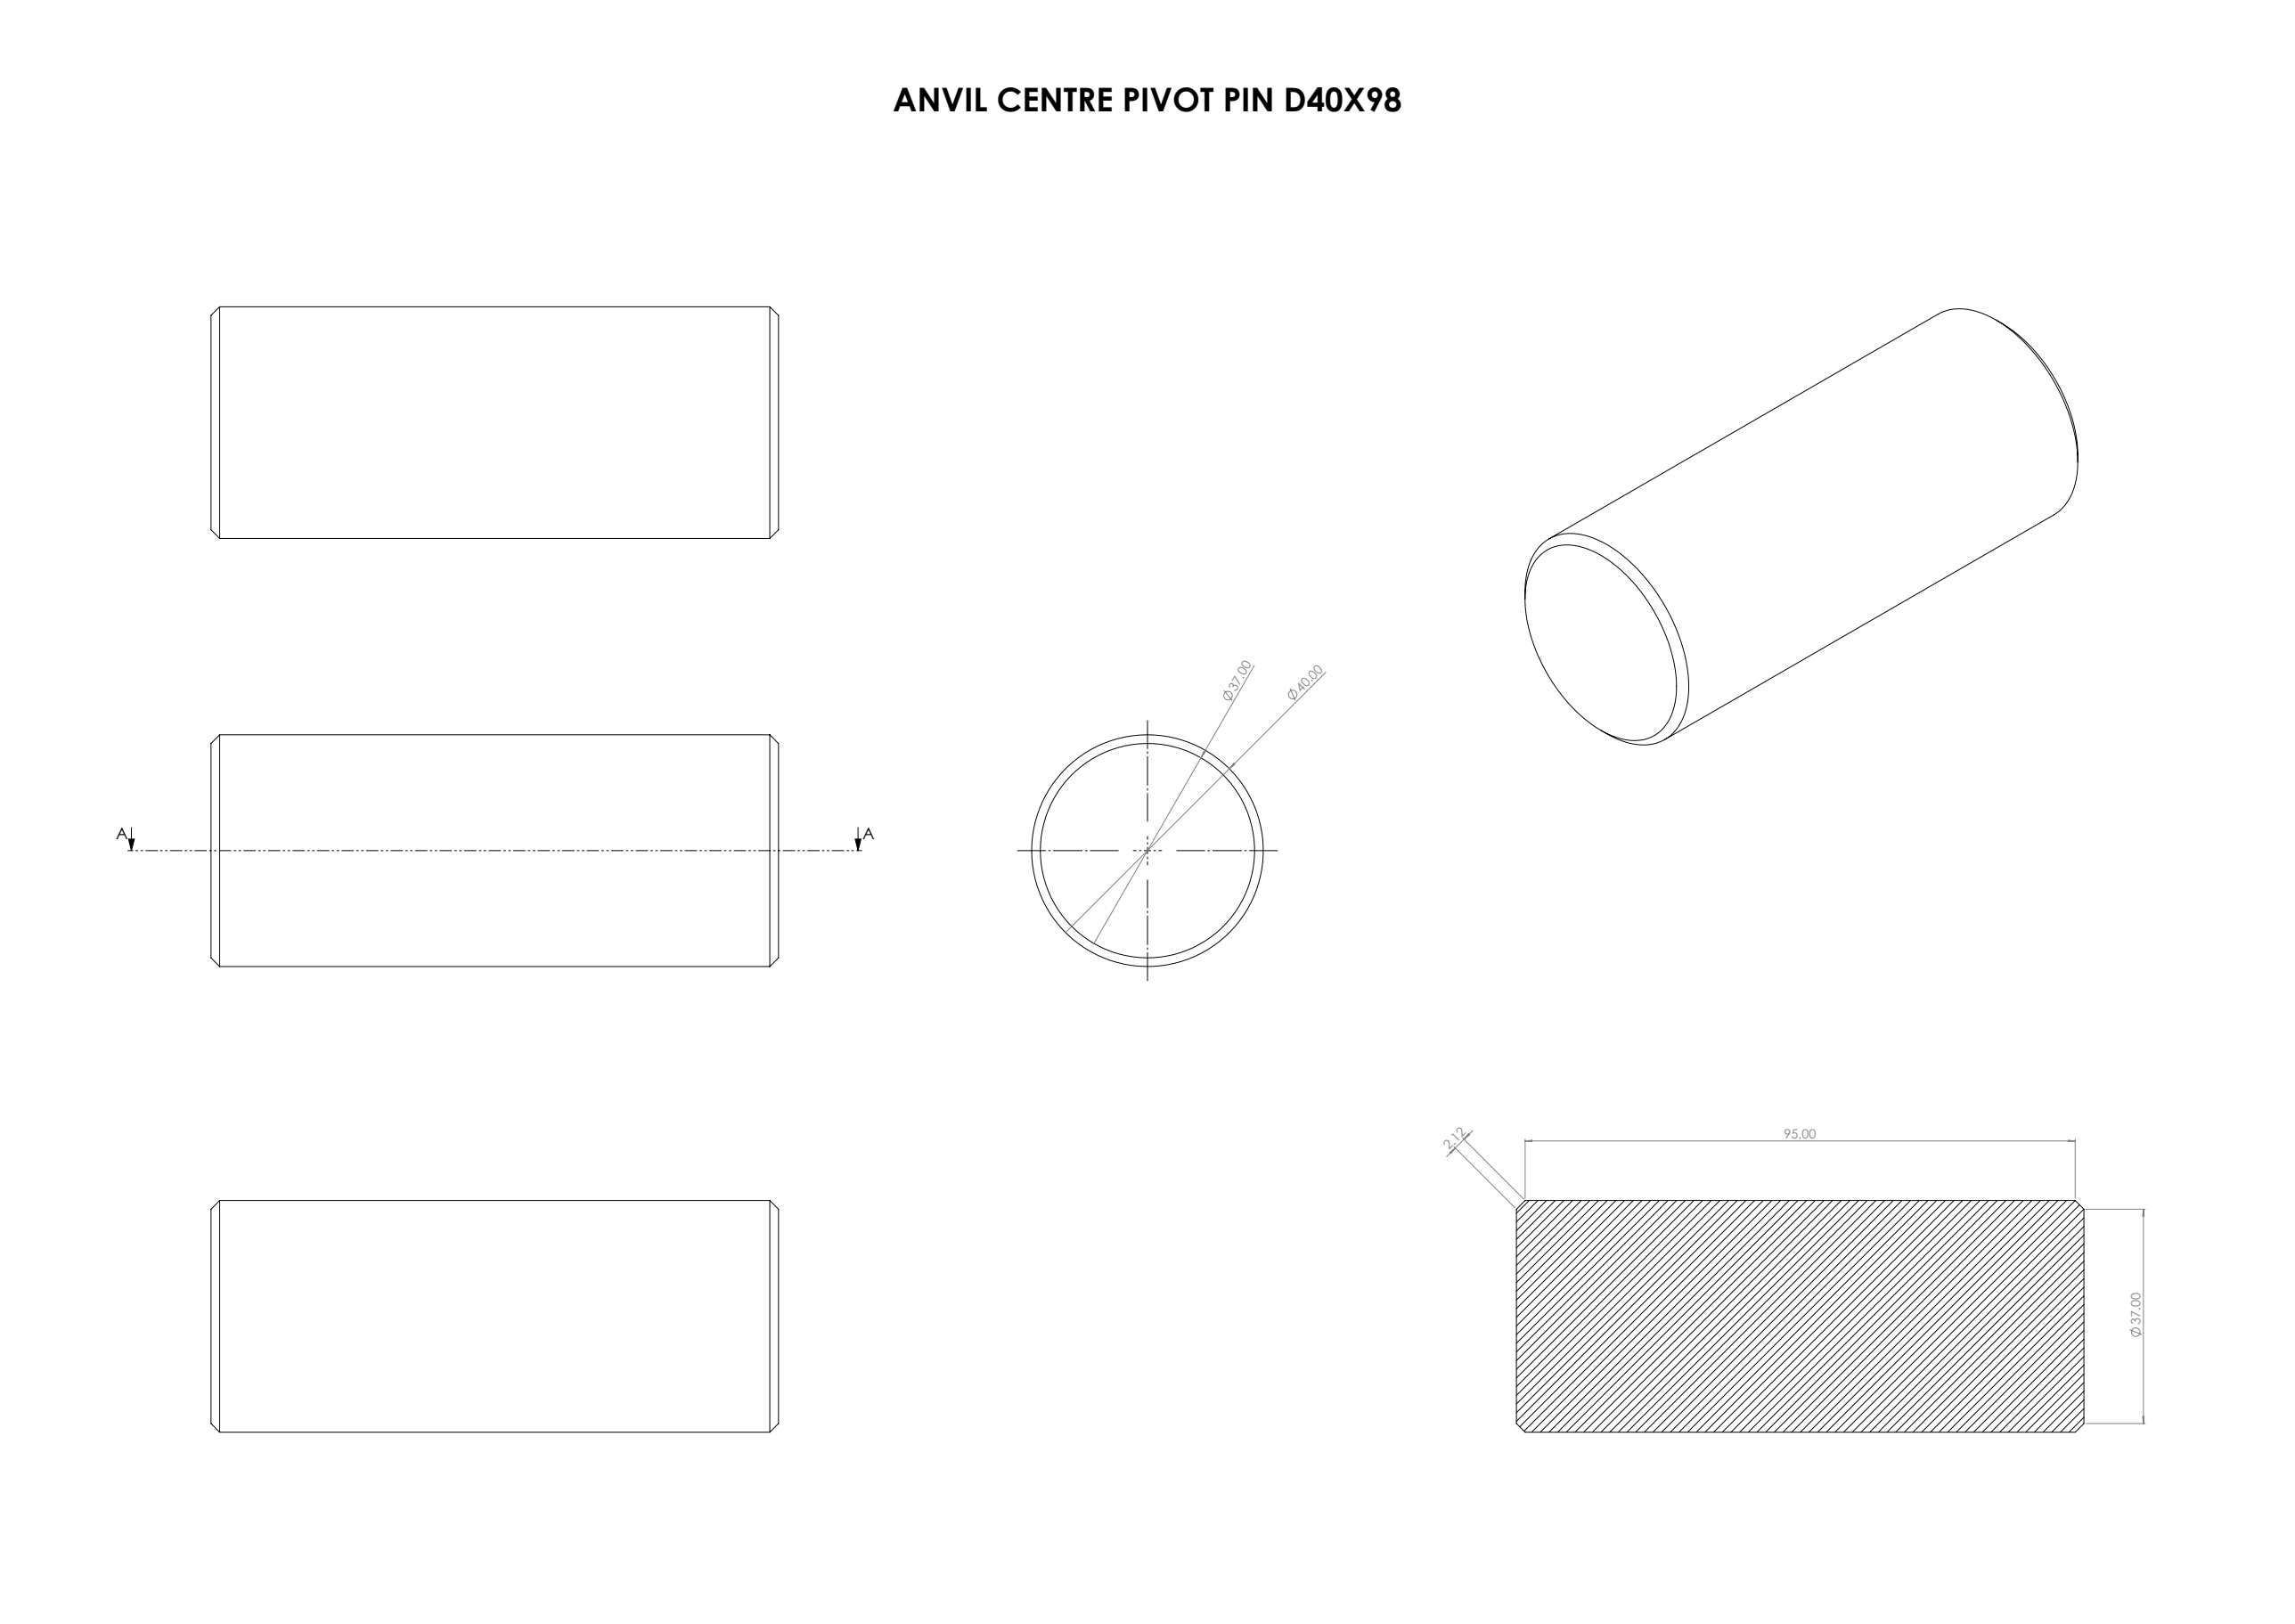
ISO-10303-21;
HEADER;
/* Generated by software containing ST-Developer
 * from STEP Tools, Inc. (www.steptools.com) 
 */

FILE_DESCRIPTION(
/* description */ (''),
/* implementation_level */ '2;1');

FILE_NAME(
/* name */ '09_Anvil_Centre_Pivot_Pin_D40x98.step',
/* time_stamp */ '2026-10-19T23:58:09-07:00',
/* author */ (''),
/* organization */ (''),
/* preprocessor_version */ 'ST-DEVELOPER v20.2',
/* originating_system */ 'Autodesk Translation Framework v15.15.0.0',
/* authorisation */ '');

FILE_SCHEMA (('AP203_CONFIGURATION_CONTROLLED_3D_DESIGN_OF_MECHANICAL_PARTS_AND_ASSEMBLIES_MIM_LF { 1 0 10303 203 3 1 4 }',
'AUTOMOTIVE_DESIGN { 1 0 10303 214 3 1 1 }','INTEGRATED_CNC_SCHEMA','MODEL_BASED_INTEGRATED_MANUFACTURING_SCHEMA',
'PROCESS_PLANNING_SCHEMA','AP242_MANAGED_MODEL_BASED_3D_ENGINEERING_MIM_LF { 1 0 10303 442 3 1 4 }'));
ENDSEC;

DATA;
#10=MECHANICAL_DESIGN_GEOMETRIC_PRESENTATION_REPRESENTATION('',(#410),#70757);
#380=SHAPE_REPRESENTATION_RELATIONSHIP('SRR','None',#70821,#395);
#395=ADVANCED_BREP_SHAPE_REPRESENTATION('',(#470),#70745);
#410=STYLED_ITEM('',(#71047),#470);
#470=MANIFOLD_SOLID_BREP('Pin',#26875);
#596=CYLINDRICAL_SURFACE('',#27394,2.);
#1761=PLANE('',#27390);
#1762=PLANE('',#27398);
#2798=FACE_OUTER_BOUND('',#4294,.T.);
#2799=FACE_OUTER_BOUND('',#4295,.T.);
#2800=FACE_OUTER_BOUND('',#4296,.T.);
#2801=FACE_OUTER_BOUND('',#4297,.T.);
#2802=FACE_OUTER_BOUND('',#4298,.T.);
#4294=EDGE_LOOP('',(#18746));
#4295=EDGE_LOOP('',(#18747,#18748,#18749,#18750));
#4296=EDGE_LOOP('',(#18751,#18752,#18753,#18754));
#4297=EDGE_LOOP('',(#18755,#18756,#18757,#18758));
#4298=EDGE_LOOP('',(#18759));
#5905=LINE('',#44061,#8402);
#5906=LINE('',#44065,#8403);
#5907=LINE('',#44069,#8404);
#8402=VECTOR('',#29942,1.925);
#8403=VECTOR('',#29947,2.);
#8404=VECTOR('',#29952,1.925);
#10766=CIRCLE('',#27391,1.85);
#10767=CIRCLE('',#27393,2.);
#10768=CIRCLE('',#27395,2.);
#10769=CIRCLE('',#27397,1.85);
#11546=VERTEX_POINT('',#44056);
#11547=VERTEX_POINT('',#44059);
#11548=VERTEX_POINT('',#44063);
#11549=VERTEX_POINT('',#44067);
#14226=EDGE_CURVE('',#11546,#11546,#10766,.T.);
#14227=EDGE_CURVE('',#11547,#11547,#10767,.T.);
#14228=EDGE_CURVE('',#11547,#11546,#5905,.T.);
#14229=EDGE_CURVE('',#11548,#11548,#10768,.T.);
#14230=EDGE_CURVE('',#11548,#11547,#5906,.T.);
#14231=EDGE_CURVE('',#11549,#11549,#10769,.T.);
#14232=EDGE_CURVE('',#11549,#11548,#5907,.T.);
#18746=ORIENTED_EDGE('',*,*,#14226,.F.);
#18747=ORIENTED_EDGE('',*,*,#14227,.F.);
#18748=ORIENTED_EDGE('',*,*,#14228,.T.);
#18749=ORIENTED_EDGE('',*,*,#14226,.T.);
#18750=ORIENTED_EDGE('',*,*,#14228,.F.);
#18751=ORIENTED_EDGE('',*,*,#14229,.F.);
#18752=ORIENTED_EDGE('',*,*,#14230,.T.);
#18753=ORIENTED_EDGE('',*,*,#14227,.T.);
#18754=ORIENTED_EDGE('',*,*,#14230,.F.);
#18755=ORIENTED_EDGE('',*,*,#14231,.F.);
#18756=ORIENTED_EDGE('',*,*,#14232,.T.);
#18757=ORIENTED_EDGE('',*,*,#14229,.T.);
#18758=ORIENTED_EDGE('',*,*,#14232,.F.);
#18759=ORIENTED_EDGE('',*,*,#14231,.T.);
#25321=CONICAL_SURFACE('',#27392,1.925,0.785398163397448);
#25322=CONICAL_SURFACE('',#27396,1.925,0.785398163397448);
#25611=ADVANCED_FACE('',(#2798),#1761,.T.);
#25612=ADVANCED_FACE('',(#2799),#25321,.T.);
#25613=ADVANCED_FACE('',(#2800),#596,.T.);
#25614=ADVANCED_FACE('',(#2801),#25322,.T.);
#25615=ADVANCED_FACE('',(#2802),#1762,.T.);
#26875=CLOSED_SHELL('',(#25611,#25612,#25613,#25614,#25615));
#27389=AXIS2_PLACEMENT_3D('',#44054,#29932,#29933);
#27390=AXIS2_PLACEMENT_3D('',#44055,#29934,#29935);
#27391=AXIS2_PLACEMENT_3D('',#44057,#29936,#29937);
#27392=AXIS2_PLACEMENT_3D('',#44058,#29938,#29939);
#27393=AXIS2_PLACEMENT_3D('',#44060,#29940,#29941);
#27394=AXIS2_PLACEMENT_3D('',#44062,#29943,#29944);
#27395=AXIS2_PLACEMENT_3D('',#44064,#29945,#29946);
#27396=AXIS2_PLACEMENT_3D('',#44066,#29948,#29949);
#27397=AXIS2_PLACEMENT_3D('',#44068,#29950,#29951);
#27398=AXIS2_PLACEMENT_3D('',#44070,#29953,#29954);
#29932=DIRECTION('axis',(0.,0.,1.));
#29933=DIRECTION('refdir',(1.,0.,0.));
#29934=DIRECTION('center_axis',(0.,0.,-1.));
#29935=DIRECTION('ref_axis',(-1.,0.,0.));
#29936=DIRECTION('center_axis',(0.,0.,1.));
#29937=DIRECTION('ref_axis',(1.,0.,0.));
#29938=DIRECTION('center_axis',(0.,0.,1.));
#29939=DIRECTION('ref_axis',(1.,0.,0.));
#29940=DIRECTION('center_axis',(0.,0.,1.));
#29941=DIRECTION('ref_axis',(1.,0.,0.));
#29942=DIRECTION('',(0.707106781186547,8.65956056235493E-17,-0.707106781186547));
#29943=DIRECTION('center_axis',(0.,0.,1.));
#29944=DIRECTION('ref_axis',(1.,0.,0.));
#29945=DIRECTION('center_axis',(0.,0.,1.));
#29946=DIRECTION('ref_axis',(1.,0.,0.));
#29947=DIRECTION('',(0.,0.,-1.));
#29948=DIRECTION('center_axis',(0.,0.,-1.));
#29949=DIRECTION('ref_axis',(1.,0.,0.));
#29950=DIRECTION('center_axis',(0.,0.,1.));
#29951=DIRECTION('ref_axis',(1.,0.,0.));
#29952=DIRECTION('',(-0.707106781186547,-8.65956056235493E-17,-0.707106781186547));
#29953=DIRECTION('center_axis',(0.,0.,1.));
#29954=DIRECTION('ref_axis',(1.,0.,0.));
#44054=CARTESIAN_POINT('',(0.,0.,0.));
#44055=CARTESIAN_POINT('Origin',(9.35,0.,5.5));
#44056=CARTESIAN_POINT('',(5.65,-2.2655965784226E-16,5.5));
#44057=CARTESIAN_POINT('Origin',(7.5,0.,5.5));
#44058=CARTESIAN_POINT('Origin',(7.5,0.,5.575));
#44059=CARTESIAN_POINT('',(5.5,-2.44929359829471E-16,5.65));
#44060=CARTESIAN_POINT('Origin',(7.5,0.,5.65));
#44061=CARTESIAN_POINT('',(5.575,-2.35744508835866E-16,5.575));
#44062=CARTESIAN_POINT('Origin',(7.5,0.,10.4));
#44063=CARTESIAN_POINT('',(5.5,-2.44929359829471E-16,15.15));
#44064=CARTESIAN_POINT('Origin',(7.5,0.,15.15));
#44065=CARTESIAN_POINT('',(5.5,-2.44929359829471E-16,10.4));
#44066=CARTESIAN_POINT('Origin',(7.5,0.,15.225));
#44067=CARTESIAN_POINT('',(5.65,-2.2655965784226E-16,15.3));
#44068=CARTESIAN_POINT('Origin',(7.5,0.,15.3));
#44069=CARTESIAN_POINT('',(5.575,-2.35744508835866E-16,15.225));
#44070=CARTESIAN_POINT('Origin',(7.5,0.,15.3));
#70728=UNCERTAINTY_MEASURE_WITH_UNIT(LENGTH_MEASURE(0.001),#70758,
'DISTANCE_ACCURACY_VALUE',
'Maximum model space distance between geometric entities at asserted c
onnectivities');
#70740=UNCERTAINTY_MEASURE_WITH_UNIT(LENGTH_MEASURE(0.001),#70758,
'DISTANCE_ACCURACY_VALUE',
'Maximum model space distance between geometric entities at asserted c
onnectivities');
#70745=(
GEOMETRIC_REPRESENTATION_CONTEXT(3)
GLOBAL_UNCERTAINTY_ASSIGNED_CONTEXT((#70728))
GLOBAL_UNIT_ASSIGNED_CONTEXT((#70758,#70760,#70761))
REPRESENTATION_CONTEXT('','3D')
);
#70757=(
GEOMETRIC_REPRESENTATION_CONTEXT(3)
GLOBAL_UNCERTAINTY_ASSIGNED_CONTEXT((#70740))
GLOBAL_UNIT_ASSIGNED_CONTEXT((#70758,#70760,#70761))
REPRESENTATION_CONTEXT('','3D')
);
#70758=(
LENGTH_UNIT()
NAMED_UNIT(*)
SI_UNIT(.CENTI.,.METRE.)
);
#70760=(
NAMED_UNIT(*)
PLANE_ANGLE_UNIT()
SI_UNIT($,.RADIAN.)
);
#70761=(
NAMED_UNIT(*)
SI_UNIT($,.STERADIAN.)
SOLID_ANGLE_UNIT()
);
#70766=SHAPE_DEFINITION_REPRESENTATION(#70782,#70821);
#70782=PRODUCT_DEFINITION_SHAPE('',$,#70838);
#70821=SHAPE_REPRESENTATION('',(#27389),#70745);
#70833=PRODUCT_DEFINITION_CONTEXT('part definition',#70883,'design');
#70838=PRODUCT_DEFINITION('2026-10-19-02-55-36-383',
'09_Anvil_Centre_Pivot_Pin_D40x98',#70854,#70833);
#70854=PRODUCT_DEFINITION_FORMATION('',$,#70889);
#70883=APPLICATION_CONTEXT(
'Core Data for Automotive Mechanical Design Process');
#70884=PRODUCT_CONTEXT('part definition',#70883,'mechanical');
#70889=PRODUCT('2026-10-19-02-55-36-383',
'09_Anvil_Centre_Pivot_Pin_D40x98',$,(#70884));
#71041=COLOUR_RGB('Grey',0.48,0.52,0.57);
#71042=FILL_AREA_STYLE_COLOUR('',#71041);
#71043=FILL_AREA_STYLE('',(#71042));
#71044=SURFACE_STYLE_FILL_AREA(#71043);
#71045=SURFACE_SIDE_STYLE('',(#71044));
#71046=SURFACE_STYLE_USAGE(.BOTH.,#71045);
#71047=PRESENTATION_STYLE_ASSIGNMENT((#71046));
ENDSEC;
END-ISO-10303-21;
